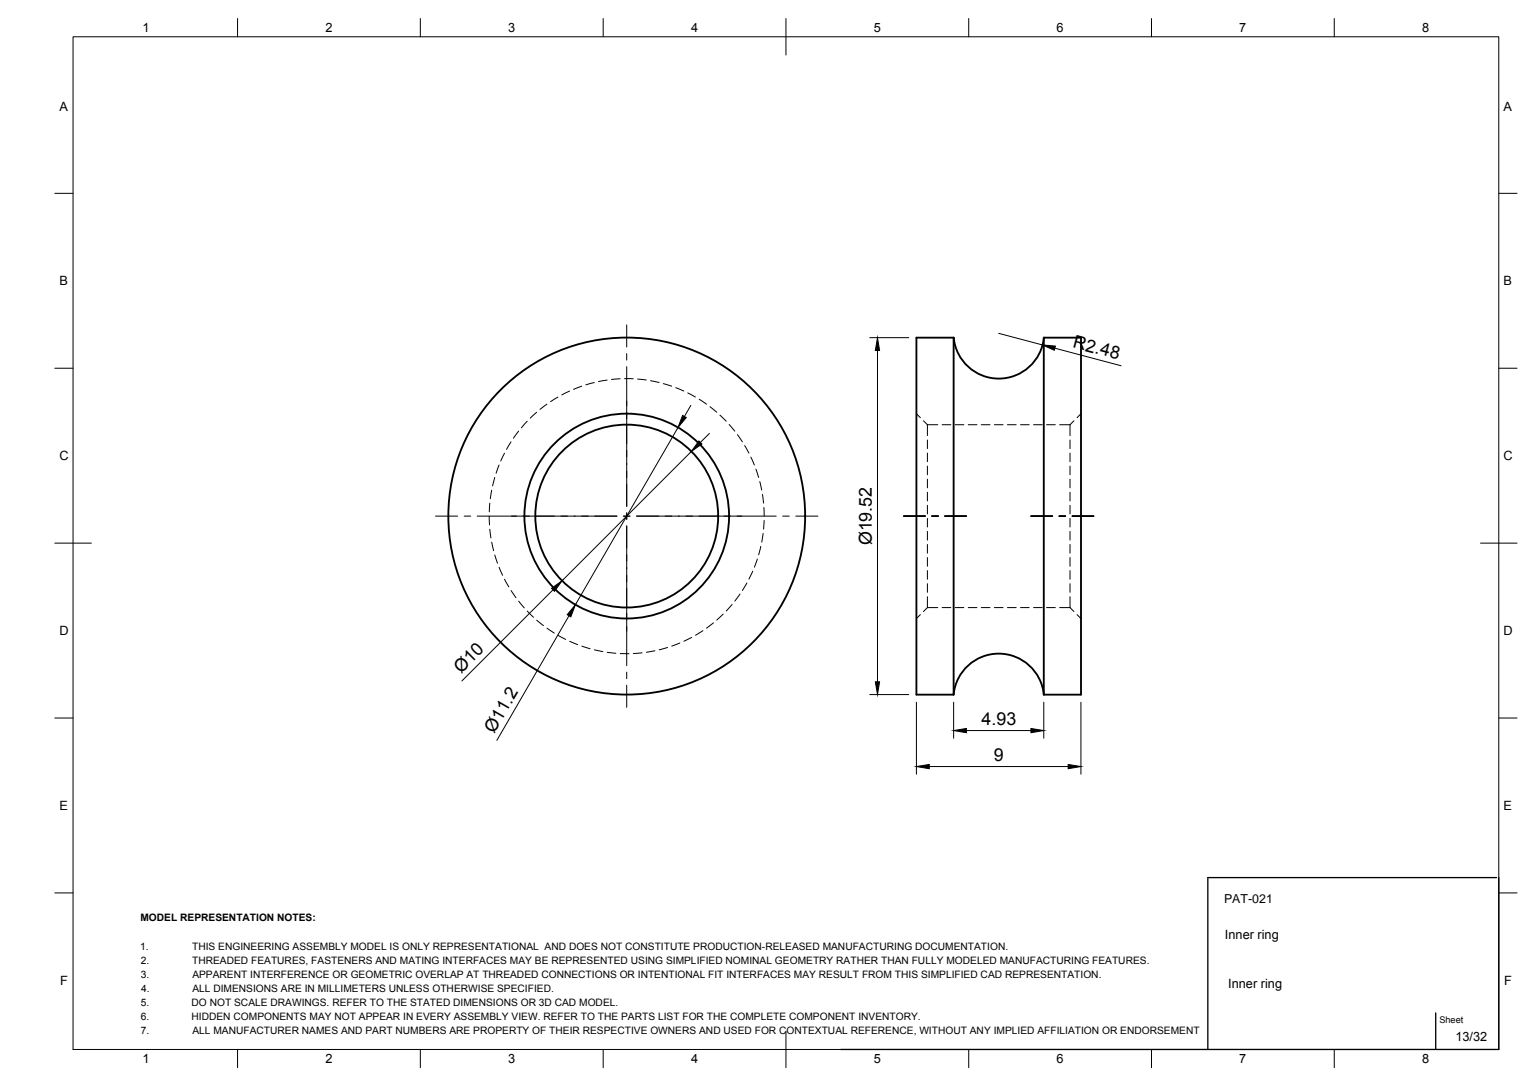
ISO-10303-21;
HEADER;
/* Generated by software containing ST-Developer
 * from STEP Tools, Inc. (www.steptools.com) 
 */

FILE_DESCRIPTION(
/* description */ ('Chain-less indexing wheel (Geneva) drive'),
/* implementation_level */ '2;1');

FILE_NAME(
/* name */ 'Inner ring.step',
/* time_stamp */ '2026-10-28T03:25:22-07:00',
/* author */ (''),
/* organization */ (''),
/* preprocessor_version */ 'ST-DEVELOPER v20.2',
/* originating_system */ 'Autodesk Translation Framework v15.17.0.0',
/* authorisation */ '');

FILE_SCHEMA (('AUTOMOTIVE_DESIGN { 1 0 10303 214 3 1 1 }'));
ENDSEC;

DATA;
#10=MECHANICAL_DESIGN_GEOMETRIC_PRESENTATION_REPRESENTATION('',(#310),#10957);
#195=TOROIDAL_SURFACE('',#6272,1.,0.247676);
#203=CONICAL_SURFACE('',#6283,0.53,0.785398163397448);
#204=CONICAL_SURFACE('',#6290,0.53,0.785398163397448);
#260=SHAPE_REPRESENTATION_RELATIONSHIP('SRR','None',#11074,#285);
#285=ADVANCED_BREP_SHAPE_REPRESENTATION('',(#342),#10937);
#310=STYLED_ITEM('',(#11287),#342);
#342=MANIFOLD_SOLID_BREP('Body1',#5707);
#424=FACE_BOUND('',#1172,.T.);
#425=FACE_BOUND('',#1175,.T.);
#539=PLANE('',#6285);
#540=PLANE('',#6288);
#777=FACE_OUTER_BOUND('',#1167,.T.);
#778=FACE_OUTER_BOUND('',#1168,.T.);
#779=FACE_OUTER_BOUND('',#1169,.T.);
#780=FACE_OUTER_BOUND('',#1170,.T.);
#781=FACE_OUTER_BOUND('',#1171,.T.);
#782=FACE_OUTER_BOUND('',#1173,.T.);
#783=FACE_OUTER_BOUND('',#1174,.T.);
#784=FACE_OUTER_BOUND('',#1176,.T.);
#1167=EDGE_LOOP('',(#4299,#4300,#4301,#4302,#4303,#4304));
#1168=EDGE_LOOP('',(#4305,#4306,#4307,#4308,#4309));
#1169=EDGE_LOOP('',(#4310,#4311,#4312,#4313));
#1170=EDGE_LOOP('',(#4314,#4315,#4316,#4317));
#1171=EDGE_LOOP('',(#4318));
#1172=EDGE_LOOP('',(#4319));
#1173=EDGE_LOOP('',(#4320,#4321,#4322,#4323,#4324));
#1174=EDGE_LOOP('',(#4325));
#1175=EDGE_LOOP('',(#4326));
#1176=EDGE_LOOP('',(#4327,#4328,#4329,#4330));
#1571=LINE('',#9263,#1945);
#1572=LINE('',#9269,#1946);
#1573=LINE('',#9273,#1947);
#1574=LINE('',#9279,#1948);
#1575=LINE('',#9284,#1949);
#1945=VECTOR('',#7435,0.976185);
#1946=VECTOR('',#7442,0.5);
#1947=VECTOR('',#7447,0.53);
#1948=VECTOR('',#7456,0.976185);
#1949=VECTOR('',#7463,0.53);
#2297=CIRCLE('',#6273,0.976185);
#2298=CIRCLE('',#6274,0.976185);
#2299=CIRCLE('',#6275,0.247676);
#2300=CIRCLE('',#6276,0.976185);
#2301=CIRCLE('',#6277,0.976185);
#2302=CIRCLE('',#6279,0.976185);
#2303=CIRCLE('',#6281,0.5);
#2304=CIRCLE('',#6282,0.5);
#2305=CIRCLE('',#6284,0.56);
#2306=CIRCLE('',#6287,0.976185);
#2307=CIRCLE('',#6289,0.56);
#2677=VERTEX_POINT('',#9252);
#2678=VERTEX_POINT('',#9253);
#2679=VERTEX_POINT('',#9256);
#2680=VERTEX_POINT('',#9258);
#2681=VERTEX_POINT('',#9262);
#2682=VERTEX_POINT('',#9266);
#2683=VERTEX_POINT('',#9268);
#2684=VERTEX_POINT('',#9272);
#2685=VERTEX_POINT('',#9277);
#2686=VERTEX_POINT('',#9281);
#3275=EDGE_CURVE('',#2677,#2678,#2297,.T.);
#3276=EDGE_CURVE('',#2678,#2677,#2298,.T.);
#3277=EDGE_CURVE('',#2678,#2679,#2299,.T.);
#3278=EDGE_CURVE('',#2680,#2679,#2300,.T.);
#3279=EDGE_CURVE('',#2679,#2680,#2301,.T.);
#3280=EDGE_CURVE('',#2680,#2681,#1571,.T.);
#3281=EDGE_CURVE('',#2681,#2681,#2302,.T.);
#3282=EDGE_CURVE('',#2682,#2682,#2303,.T.);
#3283=EDGE_CURVE('',#2682,#2683,#1572,.T.);
#3284=EDGE_CURVE('',#2683,#2683,#2304,.T.);
#3285=EDGE_CURVE('',#2683,#2684,#1573,.T.);
#3286=EDGE_CURVE('',#2684,#2684,#2305,.T.);
#3287=EDGE_CURVE('',#2685,#2685,#2306,.T.);
#3288=EDGE_CURVE('',#2685,#2677,#1574,.T.);
#3289=EDGE_CURVE('',#2686,#2686,#2307,.T.);
#3290=EDGE_CURVE('',#2686,#2682,#1575,.T.);
#4299=ORIENTED_EDGE('',*,*,#3275,.F.);
#4300=ORIENTED_EDGE('',*,*,#3276,.F.);
#4301=ORIENTED_EDGE('',*,*,#3277,.T.);
#4302=ORIENTED_EDGE('',*,*,#3278,.F.);
#4303=ORIENTED_EDGE('',*,*,#3279,.F.);
#4304=ORIENTED_EDGE('',*,*,#3277,.F.);
#4305=ORIENTED_EDGE('',*,*,#3278,.T.);
#4306=ORIENTED_EDGE('',*,*,#3279,.T.);
#4307=ORIENTED_EDGE('',*,*,#3280,.T.);
#4308=ORIENTED_EDGE('',*,*,#3281,.T.);
#4309=ORIENTED_EDGE('',*,*,#3280,.F.);
#4310=ORIENTED_EDGE('',*,*,#3282,.T.);
#4311=ORIENTED_EDGE('',*,*,#3283,.T.);
#4312=ORIENTED_EDGE('',*,*,#3284,.F.);
#4313=ORIENTED_EDGE('',*,*,#3283,.F.);
#4314=ORIENTED_EDGE('',*,*,#3284,.T.);
#4315=ORIENTED_EDGE('',*,*,#3285,.T.);
#4316=ORIENTED_EDGE('',*,*,#3286,.F.);
#4317=ORIENTED_EDGE('',*,*,#3285,.F.);
#4318=ORIENTED_EDGE('',*,*,#3281,.F.);
#4319=ORIENTED_EDGE('',*,*,#3286,.T.);
#4320=ORIENTED_EDGE('',*,*,#3287,.F.);
#4321=ORIENTED_EDGE('',*,*,#3288,.T.);
#4322=ORIENTED_EDGE('',*,*,#3275,.T.);
#4323=ORIENTED_EDGE('',*,*,#3276,.T.);
#4324=ORIENTED_EDGE('',*,*,#3288,.F.);
#4325=ORIENTED_EDGE('',*,*,#3287,.T.);
#4326=ORIENTED_EDGE('',*,*,#3289,.F.);
#4327=ORIENTED_EDGE('',*,*,#3289,.T.);
#4328=ORIENTED_EDGE('',*,*,#3290,.T.);
#4329=ORIENTED_EDGE('',*,*,#3282,.F.);
#4330=ORIENTED_EDGE('',*,*,#3290,.F.);
#5297=CYLINDRICAL_SURFACE('',#6278,0.976185);
#5298=CYLINDRICAL_SURFACE('',#6280,0.5);
#5299=CYLINDRICAL_SURFACE('',#6286,0.976185);
#5491=ADVANCED_FACE('',(#777),#195,.F.);
#5492=ADVANCED_FACE('',(#778),#5297,.T.);
#5493=ADVANCED_FACE('',(#779),#5298,.F.);
#5494=ADVANCED_FACE('',(#780),#203,.F.);
#5495=ADVANCED_FACE('',(#781,#424),#539,.T.);
#5496=ADVANCED_FACE('',(#782),#5299,.T.);
#5497=ADVANCED_FACE('',(#783,#425),#540,.T.);
#5498=ADVANCED_FACE('',(#784),#204,.F.);
#5707=CLOSED_SHELL('',(#5491,#5492,#5493,#5494,#5495,#5496,#5497,#5498));
#6271=AXIS2_PLACEMENT_3D('',#9250,#7419,#7420);
#6272=AXIS2_PLACEMENT_3D('',#9251,#7421,#7422);
#6273=AXIS2_PLACEMENT_3D('',#9254,#7423,#7424);
#6274=AXIS2_PLACEMENT_3D('',#9255,#7425,#7426);
#6275=AXIS2_PLACEMENT_3D('',#9257,#7427,#7428);
#6276=AXIS2_PLACEMENT_3D('',#9259,#7429,#7430);
#6277=AXIS2_PLACEMENT_3D('',#9260,#7431,#7432);
#6278=AXIS2_PLACEMENT_3D('',#9261,#7433,#7434);
#6279=AXIS2_PLACEMENT_3D('',#9264,#7436,#7437);
#6280=AXIS2_PLACEMENT_3D('',#9265,#7438,#7439);
#6281=AXIS2_PLACEMENT_3D('',#9267,#7440,#7441);
#6282=AXIS2_PLACEMENT_3D('',#9270,#7443,#7444);
#6283=AXIS2_PLACEMENT_3D('',#9271,#7445,#7446);
#6284=AXIS2_PLACEMENT_3D('',#9274,#7448,#7449);
#6285=AXIS2_PLACEMENT_3D('',#9275,#7450,#7451);
#6286=AXIS2_PLACEMENT_3D('',#9276,#7452,#7453);
#6287=AXIS2_PLACEMENT_3D('',#9278,#7454,#7455);
#6288=AXIS2_PLACEMENT_3D('',#9280,#7457,#7458);
#6289=AXIS2_PLACEMENT_3D('',#9282,#7459,#7460);
#6290=AXIS2_PLACEMENT_3D('',#9283,#7461,#7462);
#7419=DIRECTION('axis',(0.,0.,1.));
#7420=DIRECTION('refdir',(1.,0.,0.));
#7421=DIRECTION('center_axis',(0.,-1.,0.));
#7422=DIRECTION('ref_axis',(0.,0.,-1.));
#7423=DIRECTION('center_axis',(0.,-1.,0.));
#7424=DIRECTION('ref_axis',(1.,0.,0.));
#7425=DIRECTION('center_axis',(0.,-1.,0.));
#7426=DIRECTION('ref_axis',(1.,0.,0.));
#7427=DIRECTION('center_axis',(1.,0.,1.22464679914735E-16));
#7428=DIRECTION('ref_axis',(-1.22464679914735E-16,0.,1.));
#7429=DIRECTION('center_axis',(0.,1.,0.));
#7430=DIRECTION('ref_axis',(1.,0.,0.));
#7431=DIRECTION('center_axis',(0.,1.,0.));
#7432=DIRECTION('ref_axis',(1.,0.,0.));
#7433=DIRECTION('center_axis',(0.,-1.,0.));
#7434=DIRECTION('ref_axis',(1.,0.,0.));
#7435=DIRECTION('',(0.,1.,0.));
#7436=DIRECTION('center_axis',(0.,-1.,0.));
#7437=DIRECTION('ref_axis',(1.,0.,0.));
#7438=DIRECTION('center_axis',(0.,-1.,0.));
#7439=DIRECTION('ref_axis',(1.,0.,0.));
#7440=DIRECTION('center_axis',(0.,-1.,0.));
#7441=DIRECTION('ref_axis',(1.,0.,0.));
#7442=DIRECTION('',(0.,1.,0.));
#7443=DIRECTION('center_axis',(0.,-1.,0.));
#7444=DIRECTION('ref_axis',(1.,0.,0.));
#7445=DIRECTION('center_axis',(0.,1.,0.));
#7446=DIRECTION('ref_axis',(1.,0.,0.));
#7447=DIRECTION('',(-0.707106781186547,0.707106781186548,-8.65956056235493E-17));
#7448=DIRECTION('center_axis',(0.,-1.,0.));
#7449=DIRECTION('ref_axis',(1.,0.,0.));
#7450=DIRECTION('center_axis',(0.,1.,0.));
#7451=DIRECTION('ref_axis',(0.,0.,1.));
#7452=DIRECTION('center_axis',(0.,-1.,0.));
#7453=DIRECTION('ref_axis',(1.,0.,0.));
#7454=DIRECTION('center_axis',(0.,-1.,0.));
#7455=DIRECTION('ref_axis',(1.,0.,0.));
#7456=DIRECTION('',(0.,1.,0.));
#7457=DIRECTION('center_axis',(0.,-1.,0.));
#7458=DIRECTION('ref_axis',(0.,0.,-1.));
#7459=DIRECTION('center_axis',(0.,-1.,0.));
#7460=DIRECTION('ref_axis',(1.,0.,0.));
#7461=DIRECTION('center_axis',(0.,-1.,0.));
#7462=DIRECTION('ref_axis',(1.,0.,0.));
#7463=DIRECTION('',(0.707106781186547,0.707106781186548,8.65956056235493E-17));
#9250=CARTESIAN_POINT('',(0.,0.,0.));
#9251=CARTESIAN_POINT('Origin',(0.,0.,0.));
#9252=CARTESIAN_POINT('',(-0.976185,-0.246528389340863,-1.19548183562566E-16));
#9253=CARTESIAN_POINT('',(-1.19548183562566E-16,-0.246528389340863,0.976185));
#9254=CARTESIAN_POINT('Origin',(0.,-0.246528389340863,0.));
#9255=CARTESIAN_POINT('Origin',(0.,-0.246528389340863,0.));
#9256=CARTESIAN_POINT('',(-1.19548183562566E-16,0.246528389340863,0.976185));
#9257=CARTESIAN_POINT('Origin',(-1.22464679914735E-16,0.,1.));
#9258=CARTESIAN_POINT('',(-0.976185,0.246528389340863,1.19548183562566E-16));
#9259=CARTESIAN_POINT('Origin',(0.,0.246528389340863,0.));
#9260=CARTESIAN_POINT('Origin',(0.,0.246528389340863,0.));
#9261=CARTESIAN_POINT('Origin',(0.,0.,0.));
#9262=CARTESIAN_POINT('',(-0.976185,0.45,-1.19548183562566E-16));
#9263=CARTESIAN_POINT('',(-0.976185,0.,-1.19548183562566E-16));
#9264=CARTESIAN_POINT('Origin',(0.,0.45,0.));
#9265=CARTESIAN_POINT('Origin',(0.,0.,0.));
#9266=CARTESIAN_POINT('',(-0.5,-0.39,-6.12323399573677E-17));
#9267=CARTESIAN_POINT('Origin',(0.,-0.39,0.));
#9268=CARTESIAN_POINT('',(-0.5,0.39,-6.12323399573677E-17));
#9269=CARTESIAN_POINT('',(-0.5,0.,-6.12323399573677E-17));
#9270=CARTESIAN_POINT('Origin',(0.,0.39,0.));
#9271=CARTESIAN_POINT('Origin',(0.,0.42,0.));
#9272=CARTESIAN_POINT('',(-0.56,0.45,-6.85802207522518E-17));
#9273=CARTESIAN_POINT('',(-0.53,0.42,-6.49062803548097E-17));
#9274=CARTESIAN_POINT('Origin',(0.,0.45,0.));
#9275=CARTESIAN_POINT('Origin',(0.976185,0.45,0.));
#9276=CARTESIAN_POINT('Origin',(0.,0.,0.));
#9277=CARTESIAN_POINT('',(-0.976185,-0.45,-1.19548183562566E-16));
#9278=CARTESIAN_POINT('Origin',(0.,-0.45,0.));
#9279=CARTESIAN_POINT('',(-0.976185,0.,-1.19548183562566E-16));
#9280=CARTESIAN_POINT('Origin',(0.56,-0.45,0.));
#9281=CARTESIAN_POINT('',(-0.56,-0.45,-6.85802207522518E-17));
#9282=CARTESIAN_POINT('Origin',(0.,-0.45,0.));
#9283=CARTESIAN_POINT('Origin',(0.,-0.42,0.));
#9284=CARTESIAN_POINT('',(-0.53,-0.42,-6.49062803548097E-17));
#10906=UNCERTAINTY_MEASURE_WITH_UNIT(LENGTH_MEASURE(0.001),#10958,
'DISTANCE_ACCURACY_VALUE',
'Maximum model space distance between geometric entities at asserted c
onnectivities');
#10926=UNCERTAINTY_MEASURE_WITH_UNIT(LENGTH_MEASURE(0.001),#10958,
'DISTANCE_ACCURACY_VALUE',
'Maximum model space distance between geometric entities at asserted c
onnectivities');
#10937=(
GEOMETRIC_REPRESENTATION_CONTEXT(3)
GLOBAL_UNCERTAINTY_ASSIGNED_CONTEXT((#10906))
GLOBAL_UNIT_ASSIGNED_CONTEXT((#10958,#10960,#10961))
REPRESENTATION_CONTEXT('','3D')
);
#10957=(
GEOMETRIC_REPRESENTATION_CONTEXT(3)
GLOBAL_UNCERTAINTY_ASSIGNED_CONTEXT((#10926))
GLOBAL_UNIT_ASSIGNED_CONTEXT((#10958,#10960,#10961))
REPRESENTATION_CONTEXT('','3D')
);
#10958=(
LENGTH_UNIT()
NAMED_UNIT(*)
SI_UNIT(.CENTI.,.METRE.)
);
#10960=(
NAMED_UNIT(*)
PLANE_ANGLE_UNIT()
SI_UNIT($,.RADIAN.)
);
#10961=(
NAMED_UNIT(*)
SI_UNIT($,.STERADIAN.)
SOLID_ANGLE_UNIT()
);
#10972=SHAPE_DEFINITION_REPRESENTATION(#11002,#11074);
#11002=PRODUCT_DEFINITION_SHAPE('',$,#11105);
#11074=SHAPE_REPRESENTATION('',(#6271),#10937);
#11094=PRODUCT_DEFINITION_CONTEXT('part definition',#11186,'design');
#11105=PRODUCT_DEFINITION('Inner ring','Inner ring',#11135,#11094);
#11135=PRODUCT_DEFINITION_FORMATION('',$,#11198);
#11186=APPLICATION_CONTEXT(
'Core Data for Automotive Mechanical Design Process');
#11187=PRODUCT_CONTEXT('part definition',#11186,'mechanical');
#11198=PRODUCT('Inner ring','Inner ring','Inner ring',(#11187));
#11281=COLOUR_RGB('Grey',0.48,0.52,0.57);
#11282=FILL_AREA_STYLE_COLOUR('',#11281);
#11283=FILL_AREA_STYLE('',(#11282));
#11284=SURFACE_STYLE_FILL_AREA(#11283);
#11285=SURFACE_SIDE_STYLE('',(#11284));
#11286=SURFACE_STYLE_USAGE(.BOTH.,#11285);
#11287=PRESENTATION_STYLE_ASSIGNMENT((#11286));
ENDSEC;
END-ISO-10303-21;
